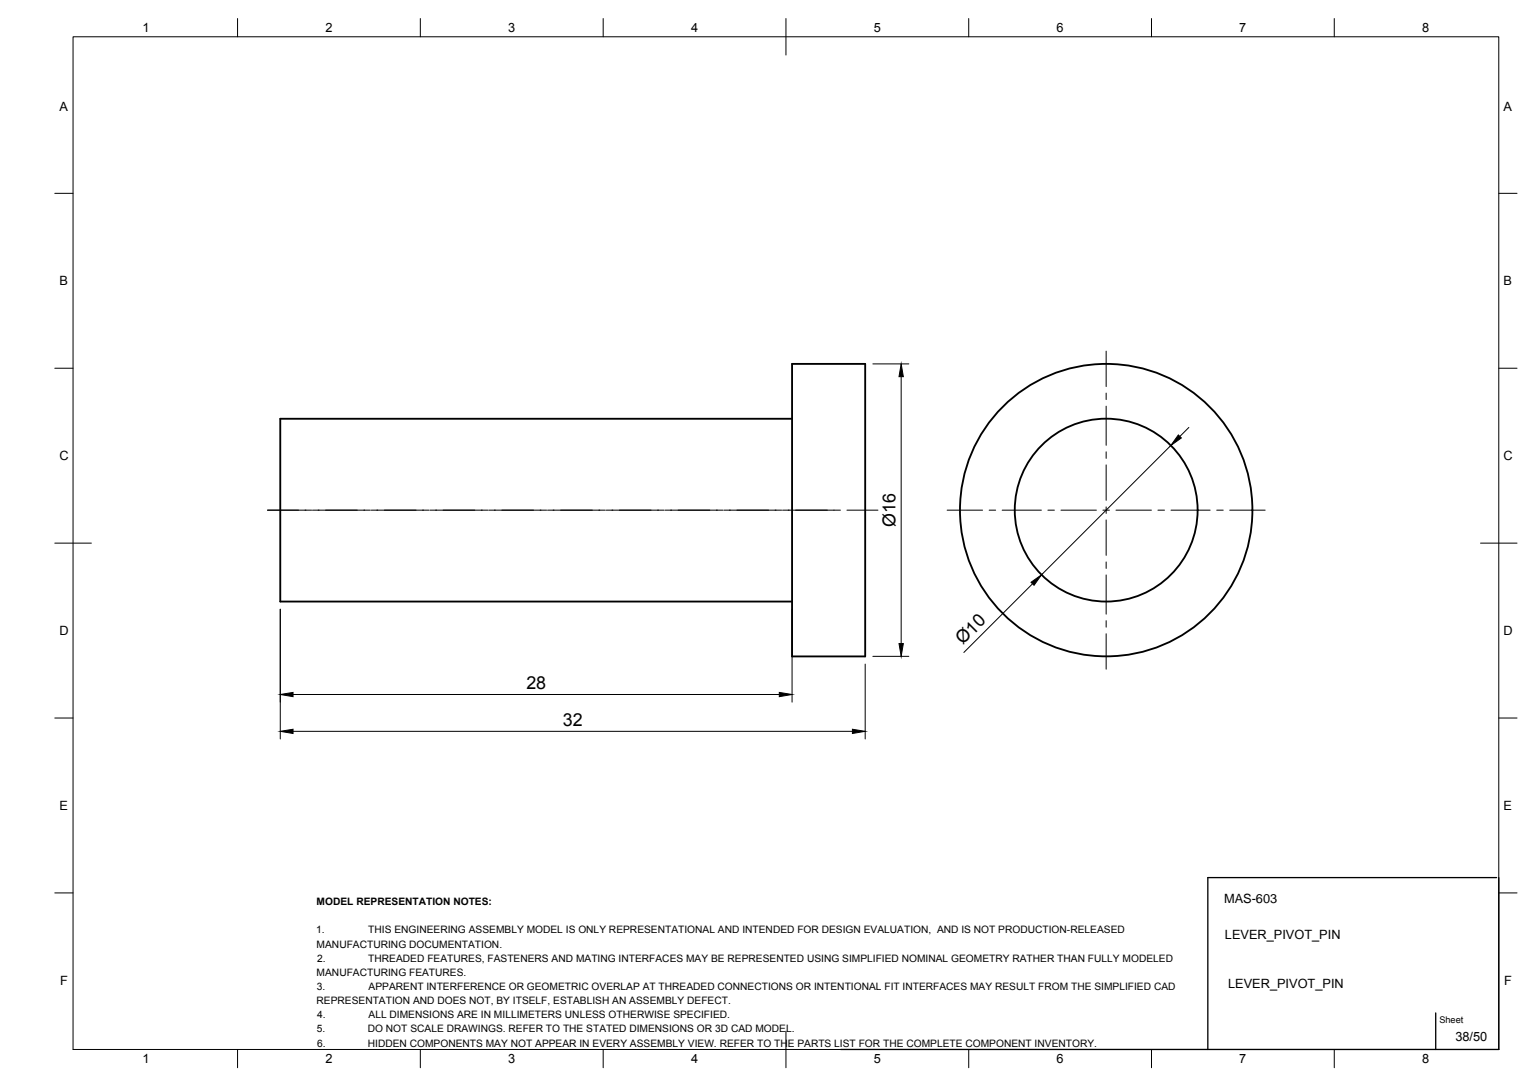
ISO-10303-21;
HEADER;
FILE_DESCRIPTION((''),'2;1');
FILE_NAME('LEVER_PIVOT_PIN.step','2026-10-01T22:06:14-07:00',(''),(''),'','','');
FILE_SCHEMA (('AUTOMOTIVE_DESIGN { 1 0 10303 214 3 1 1 }'));
ENDSEC;
DATA;
#10=MECHANICAL_DESIGN_GEOMETRIC_PRESENTATION_REPRESENTATION('',(#1011),#50440);
#918=SHAPE_REPRESENTATION_RELATIONSHIP('SRR','None',#50651,#963) ;
#963=ADVANCED_BREP_SHAPE_REPRESENTATION('',(#1066),#50420) ;
#1011=STYLED_ITEM('',(#50883),#1066) ;
#1066=MANIFOLD_SOLID_BREP('LEVER_PIVOT_PIN',#28678) ;
#1376=FACE_BOUND('',#5234,.T.) ;
#2229=PLANE('',#30933) ;
#2230=PLANE('',#30938) ;
#2231=PLANE('',#30941) ;
#3415=FACE_OUTER_BOUND('',#5233,.T.) ;
#3416=FACE_OUTER_BOUND('',#5235,.T.) ;
#3417=FACE_OUTER_BOUND('',#5236,.T.) ;
#3418=FACE_OUTER_BOUND('',#5237,.T.) ;
#3419=FACE_OUTER_BOUND('',#5238,.T.) ;
#5233=EDGE_LOOP('',(#24093)) ;
#5234=EDGE_LOOP('',(#24094)) ;
#5235=EDGE_LOOP('',(#24095,#24096,#24097,#24098)) ;
#5236=EDGE_LOOP('',(#24099)) ;
#5237=EDGE_LOOP('',(#24100,#24101,#24102,#24103)) ;
#5238=EDGE_LOOP('',(#24104)) ;
#7879=LINE('',#47193,#10351) ;
#7880=LINE('',#47199,#10352) ;
#10351=VECTOR('',#37978,0.8) ;
#10352=VECTOR('',#37987,0.5) ;
#11235=CIRCLE('',#30934,0.8) ;
#11236=CIRCLE('',#30935,0.5) ;
#11237=CIRCLE('',#30937,0.8) ;
#11238=CIRCLE('',#30940,0.5) ;
#13679=VERTEX_POINT('',#47187) ;
#13680=VERTEX_POINT('',#47189) ;
#13681=VERTEX_POINT('',#47192) ;
#13682=VERTEX_POINT('',#47197) ;
#17312=EDGE_CURVE('',#13679,#13679,#11235,.T.) ;
#17313=EDGE_CURVE('',#13680,#13680,#11236,.T.) ;
#17314=EDGE_CURVE('',#13679,#13681,#7879,.T.) ;
#17315=EDGE_CURVE('',#13681,#13681,#11237,.T.) ;
#17316=EDGE_CURVE('',#13682,#13682,#11238,.T.) ;
#17317=EDGE_CURVE('',#13682,#13680,#7880,.T.) ;
#24093=ORIENTED_EDGE('',*,*,#17312,.T.) ;
#24094=ORIENTED_EDGE('',*,*,#17313,.T.) ;
#24095=ORIENTED_EDGE('',*,*,#17312,.F.) ;
#24096=ORIENTED_EDGE('',*,*,#17314,.T.) ;
#24097=ORIENTED_EDGE('',*,*,#17315,.F.) ;
#24098=ORIENTED_EDGE('',*,*,#17314,.F.) ;
#24099=ORIENTED_EDGE('',*,*,#17315,.T.) ;
#24100=ORIENTED_EDGE('',*,*,#17316,.F.) ;
#24101=ORIENTED_EDGE('',*,*,#17317,.T.) ;
#24102=ORIENTED_EDGE('',*,*,#17313,.F.) ;
#24103=ORIENTED_EDGE('',*,*,#17317,.F.) ;
#24104=ORIENTED_EDGE('',*,*,#17316,.T.) ;
#26870=CYLINDRICAL_SURFACE('',#30936,0.8) ;
#26871=CYLINDRICAL_SURFACE('',#30939,0.5) ;
#28150=ADVANCED_FACE('',(#3415,#1376),#2229,.T.) ;
#28151=ADVANCED_FACE('',(#3416),#26870,.T.) ;
#28152=ADVANCED_FACE('',(#3417),#2230,.T.) ;
#28153=ADVANCED_FACE('',(#3418),#26871,.T.) ;
#28154=ADVANCED_FACE('',(#3419),#2231,.T.) ;
#28678=CLOSED_SHELL('',(#28150,#28151,#28152,#28153,#28154)) ;
#30932=AXIS2_PLACEMENT_3D('',#47185,#37968,#37969) ;
#30933=AXIS2_PLACEMENT_3D('',#47186,#37970,#37971) ;
#30934=AXIS2_PLACEMENT_3D('',#47188,#37972,#37973) ;
#30935=AXIS2_PLACEMENT_3D('',#47190,#37974,#37975) ;
#30936=AXIS2_PLACEMENT_3D('',#47191,#37976,#37977) ;
#30937=AXIS2_PLACEMENT_3D('',#47194,#37979,#37980) ;
#30938=AXIS2_PLACEMENT_3D('',#47195,#37981,#37982) ;
#30939=AXIS2_PLACEMENT_3D('',#47196,#37983,#37984) ;
#30940=AXIS2_PLACEMENT_3D('',#47198,#37985,#37986) ;
#30941=AXIS2_PLACEMENT_3D('',#47200,#37988,#37989) ;
#37968=DIRECTION('axis',(0.,0.,1.)) ;
#37969=DIRECTION('refdir',(1.,0.,0.)) ;
#37970=DIRECTION('center_axis',(0.,1.,0.)) ;
#37971=DIRECTION('ref_axis',(1.,0.,0.)) ;
#37972=DIRECTION('center_axis',(0.,1.,0.)) ;
#37973=DIRECTION('ref_axis',(1.,0.,0.)) ;
#37974=DIRECTION('center_axis',(0.,-1.,0.)) ;
#37975=DIRECTION('ref_axis',(1.,0.,0.)) ;
#37976=DIRECTION('center_axis',(0.,1.,0.)) ;
#37977=DIRECTION('ref_axis',(1.,0.,0.)) ;
#37978=DIRECTION('',(0.,-1.,0.)) ;
#37979=DIRECTION('center_axis',(0.,-1.,0.)) ;
#37980=DIRECTION('ref_axis',(1.,0.,0.)) ;
#37981=DIRECTION('center_axis',(0.,-1.,0.)) ;
#37982=DIRECTION('ref_axis',(-1.,0.,0.)) ;
#37983=DIRECTION('center_axis',(0.,1.,0.)) ;
#37984=DIRECTION('ref_axis',(1.,0.,0.)) ;
#37985=DIRECTION('center_axis',(0.,1.,0.)) ;
#37986=DIRECTION('ref_axis',(1.,0.,0.)) ;
#37987=DIRECTION('',(0.,-1.,0.)) ;
#37988=DIRECTION('center_axis',(0.,1.,0.)) ;
#37989=DIRECTION('ref_axis',(1.,0.,0.)) ;
#47185=CARTESIAN_POINT('',(0.,0.,0.)) ;
#47186=CARTESIAN_POINT('Origin',(-53.,17.6,92.)) ;
#47187=CARTESIAN_POINT('',(-53.8,17.6,92.)) ;
#47188=CARTESIAN_POINT('Origin',(-53.,17.6,92.)) ;
#47189=CARTESIAN_POINT('',(-53.5,17.6,92.)) ;
#47190=CARTESIAN_POINT('Origin',(-53.,17.6,92.)) ;
#47191=CARTESIAN_POINT('Origin',(-53.,17.4,92.)) ;
#47192=CARTESIAN_POINT('',(-53.8,17.2,92.)) ;
#47193=CARTESIAN_POINT('',(-53.8,17.4,92.)) ;
#47194=CARTESIAN_POINT('Origin',(-53.,17.2,92.)) ;
#47195=CARTESIAN_POINT('Origin',(-53.,17.2,92.)) ;
#47196=CARTESIAN_POINT('Origin',(-53.,19.,92.)) ;
#47197=CARTESIAN_POINT('',(-53.5,20.4,92.)) ;
#47198=CARTESIAN_POINT('Origin',(-53.,20.4,92.)) ;
#47199=CARTESIAN_POINT('',(-53.5,19.,92.)) ;
#47200=CARTESIAN_POINT('Origin',(-53.,20.4,92.)) ;
#50367=UNCERTAINTY_MEASURE_WITH_UNIT(LENGTH_MEASURE(0.001),#50441,
'DISTANCE_ACCURACY_VALUE',
'Maximum model space distance between geometric entities at asserted c
onnectivities') ;
#50387=UNCERTAINTY_MEASURE_WITH_UNIT(LENGTH_MEASURE(0.001),#50441,
'DISTANCE_ACCURACY_VALUE',
'Maximum model space distance between geometric entities at asserted c
onnectivities') ;
#50420=(
GEOMETRIC_REPRESENTATION_CONTEXT(3)
GLOBAL_UNCERTAINTY_ASSIGNED_CONTEXT((#50367))
GLOBAL_UNIT_ASSIGNED_CONTEXT((#50441,#50443,#50444))
REPRESENTATION_CONTEXT('','3D')
) ;
#50440=(
GEOMETRIC_REPRESENTATION_CONTEXT(3)
GLOBAL_UNCERTAINTY_ASSIGNED_CONTEXT((#50387))
GLOBAL_UNIT_ASSIGNED_CONTEXT((#50441,#50443,#50444))
REPRESENTATION_CONTEXT('','3D')
) ;
#50441=(
LENGTH_UNIT()
NAMED_UNIT(*)
SI_UNIT(.CENTI.,.METRE.)
) ;
#50443=(
NAMED_UNIT(*)
PLANE_ANGLE_UNIT()
SI_UNIT($,.RADIAN.)
) ;
#50444=(
NAMED_UNIT(*)
SI_UNIT($,.STERADIAN.)
SOLID_ANGLE_UNIT()
) ;
#50477=SHAPE_DEFINITION_REPRESENTATION(#50553,#50651) ;
#50553=PRODUCT_DEFINITION_SHAPE('',$,#50704) ;
#50651=SHAPE_REPRESENTATION('',(#30932),#50420) ;
#50671=PRODUCT_DEFINITION_CONTEXT('part definition',#50829,'design') ;
#50704=PRODUCT_DEFINITION('LEVER_PIVOT_PIN','LEVER_PIVOT_PIN',#50756,
#50671) ;
#50756=PRODUCT_DEFINITION_FORMATION('',$,#50863) ;
#50829=APPLICATION_CONTEXT(
'Core Data for Automotive Mechanical Design Process') ;
#50830=PRODUCT_CONTEXT('part definition',#50829,'mechanical') ;
#50863=PRODUCT('LEVER_PIVOT_PIN','LEVER_PIVOT_PIN',$,(#50830)) ;
#50883=PRESENTATION_STYLE_ASSIGNMENT((#50890)) ;
#50890=SURFACE_STYLE_USAGE(.BOTH.,#50897) ;
#50897=SURFACE_SIDE_STYLE('',(#50904)) ;
#50904=SURFACE_STYLE_FILL_AREA(#50911) ;
#50911=FILL_AREA_STYLE('Steel - Satin',(#50918)) ;
#50918=FILL_AREA_STYLE_COLOUR('Steel - Satin',#50925) ;
#50925=COLOUR_RGB('Steel - Satin', 0.31764706, 0.68627451, 0.89019608) ;
ENDSEC;
END-ISO-10303-21;
